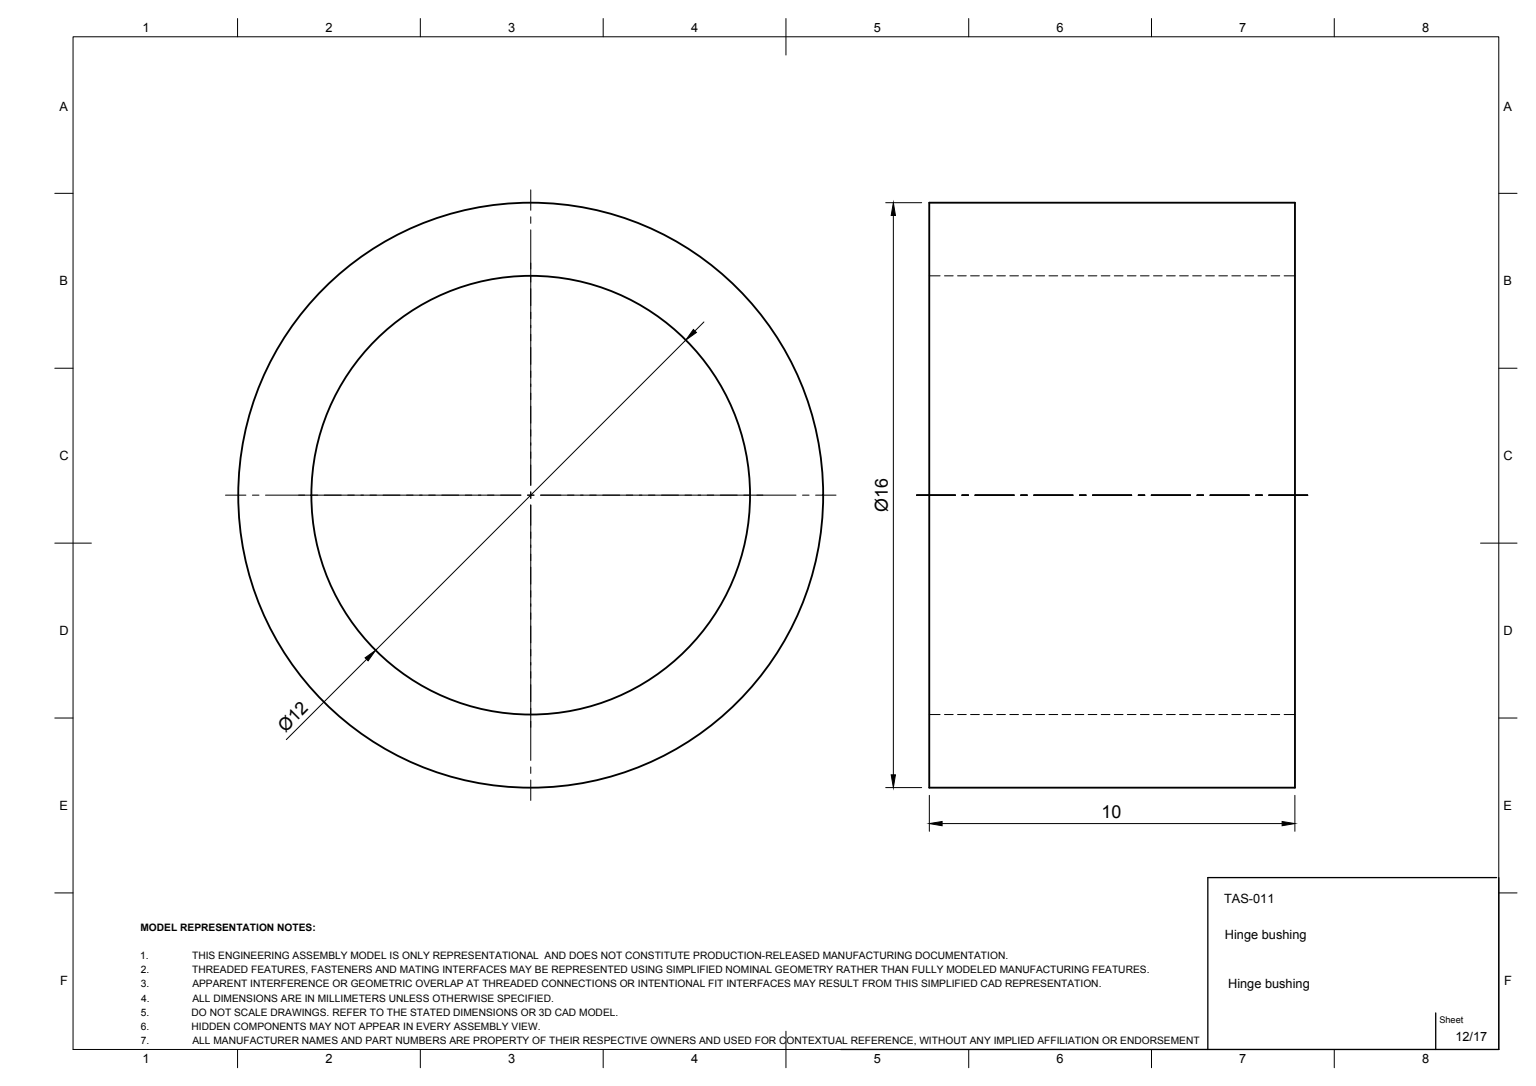
ISO-10303-21;
HEADER;
/* Generated by software containing ST-Developer
 * from STEP Tools, Inc. (www.steptools.com) 
 */

FILE_DESCRIPTION(
/* description */ (
'Independent manual bench leaf bending machine,200mm work width. Fabri
cated welded frame and folding leaf, repeated bushed and fully retaine
d hinge hardware, two handles with bonded grips, beveled clamping beam
 and modeledM12 clamp screws.2mm omitted-workpiece assembly reference 
gap, not a capacity claim. Native135deg hinge travel. Weld sizing, pro
duction fits, material condition, bending capacity, strength and life 
unassigned.'),
/* implementation_level */ '2;1');

FILE_NAME(
/* name */ 'Hinge bushing.step',
/* time_stamp */ '2026-11-14T09:11:34-08:00',
/* author */ (''),
/* organization */ (''),
/* preprocessor_version */ 'ST-DEVELOPER v20.2',
/* originating_system */ 'Autodesk Translation Framework v15.17.0.0',
/* authorisation */ '');

FILE_SCHEMA (('AUTOMOTIVE_DESIGN { 1 0 10303 214 3 1 1 }'));
ENDSEC;

DATA;
#10=MECHANICAL_DESIGN_GEOMETRIC_PRESENTATION_REPRESENTATION('',(#457),#37701);
#421=SHAPE_REPRESENTATION_RELATIONSHIP('SRR','None',#37790,#439);
#439=ADVANCED_BREP_SHAPE_REPRESENTATION('',(#475),#37694);
#457=STYLED_ITEM('',(#37880),#475);
#475=MANIFOLD_SOLID_BREP('Body1',#4155);
#508=FACE_BOUND('',#1018,.T.);
#509=FACE_BOUND('',#1020,.T.);
#578=PLANE('',#4610);
#579=PLANE('',#4611);
#777=FACE_OUTER_BOUND('',#1015,.T.);
#778=FACE_OUTER_BOUND('',#1016,.T.);
#779=FACE_OUTER_BOUND('',#1017,.T.);
#780=FACE_OUTER_BOUND('',#1019,.T.);
#1015=EDGE_LOOP('',(#3697,#3698,#3699,#3700));
#1016=EDGE_LOOP('',(#3701,#3702,#3703,#3704));
#1017=EDGE_LOOP('',(#3705));
#1018=EDGE_LOOP('',(#3706));
#1019=EDGE_LOOP('',(#3707));
#1020=EDGE_LOOP('',(#3708));
#1278=LINE('',#37494,#1527);
#1279=LINE('',#37500,#1528);
#1527=VECTOR('',#5415,6.);
#1528=VECTOR('',#5422,8.);
#1611=CIRCLE('',#4605,6.);
#1612=CIRCLE('',#4606,6.);
#1613=CIRCLE('',#4608,8.);
#1614=CIRCLE('',#4609,8.);
#2015=VERTEX_POINT('',#37491);
#2016=VERTEX_POINT('',#37493);
#2017=VERTEX_POINT('',#37497);
#2018=VERTEX_POINT('',#37499);
#2582=EDGE_CURVE('',#2015,#2015,#1611,.T.);
#2583=EDGE_CURVE('',#2015,#2016,#1278,.T.);
#2584=EDGE_CURVE('',#2016,#2016,#1612,.T.);
#2585=EDGE_CURVE('',#2017,#2017,#1613,.T.);
#2586=EDGE_CURVE('',#2017,#2018,#1279,.T.);
#2587=EDGE_CURVE('',#2018,#2018,#1614,.T.);
#3697=ORIENTED_EDGE('',*,*,#2582,.T.);
#3698=ORIENTED_EDGE('',*,*,#2583,.T.);
#3699=ORIENTED_EDGE('',*,*,#2584,.F.);
#3700=ORIENTED_EDGE('',*,*,#2583,.F.);
#3701=ORIENTED_EDGE('',*,*,#2585,.F.);
#3702=ORIENTED_EDGE('',*,*,#2586,.T.);
#3703=ORIENTED_EDGE('',*,*,#2587,.T.);
#3704=ORIENTED_EDGE('',*,*,#2586,.F.);
#3705=ORIENTED_EDGE('',*,*,#2585,.T.);
#3706=ORIENTED_EDGE('',*,*,#2584,.T.);
#3707=ORIENTED_EDGE('',*,*,#2587,.F.);
#3708=ORIENTED_EDGE('',*,*,#2582,.F.);
#3919=CYLINDRICAL_SURFACE('',#4604,6.);
#3920=CYLINDRICAL_SURFACE('',#4607,8.);
#4107=ADVANCED_FACE('',(#777),#3919,.F.);
#4108=ADVANCED_FACE('',(#778),#3920,.T.);
#4109=ADVANCED_FACE('',(#779,#508),#578,.T.);
#4110=ADVANCED_FACE('',(#780,#509),#579,.F.);
#4155=CLOSED_SHELL('',(#4107,#4108,#4109,#4110));
#4603=AXIS2_PLACEMENT_3D('',#37489,#5409,#5410);
#4604=AXIS2_PLACEMENT_3D('',#37490,#5411,#5412);
#4605=AXIS2_PLACEMENT_3D('',#37492,#5413,#5414);
#4606=AXIS2_PLACEMENT_3D('',#37495,#5416,#5417);
#4607=AXIS2_PLACEMENT_3D('',#37496,#5418,#5419);
#4608=AXIS2_PLACEMENT_3D('',#37498,#5420,#5421);
#4609=AXIS2_PLACEMENT_3D('',#37501,#5423,#5424);
#4610=AXIS2_PLACEMENT_3D('',#37502,#5425,#5426);
#4611=AXIS2_PLACEMENT_3D('',#37503,#5427,#5428);
#5409=DIRECTION('axis',(0.,0.,1.));
#5410=DIRECTION('refdir',(1.,0.,0.));
#5411=DIRECTION('center_axis',(0.,0.,1.));
#5412=DIRECTION('ref_axis',(1.,0.,0.));
#5413=DIRECTION('center_axis',(0.,0.,-1.));
#5414=DIRECTION('ref_axis',(1.,0.,0.));
#5415=DIRECTION('',(0.,0.,1.));
#5416=DIRECTION('center_axis',(0.,0.,-1.));
#5417=DIRECTION('ref_axis',(1.,0.,0.));
#5418=DIRECTION('center_axis',(0.,0.,1.));
#5419=DIRECTION('ref_axis',(1.,0.,0.));
#5420=DIRECTION('center_axis',(0.,0.,1.));
#5421=DIRECTION('ref_axis',(1.,0.,0.));
#5422=DIRECTION('',(0.,0.,-1.));
#5423=DIRECTION('center_axis',(0.,0.,1.));
#5424=DIRECTION('ref_axis',(1.,0.,0.));
#5425=DIRECTION('center_axis',(0.,0.,1.));
#5426=DIRECTION('ref_axis',(1.,0.,0.));
#5427=DIRECTION('center_axis',(0.,0.,1.));
#5428=DIRECTION('ref_axis',(1.,0.,0.));
#37489=CARTESIAN_POINT('',(0.,0.,0.));
#37490=CARTESIAN_POINT('Origin',(0.,0.,0.));
#37491=CARTESIAN_POINT('',(-6.,-7.34788079488412E-16,0.));
#37492=CARTESIAN_POINT('Origin',(0.,0.,0.));
#37493=CARTESIAN_POINT('',(-6.,-7.34788079488412E-16,10.));
#37494=CARTESIAN_POINT('',(-6.,-7.34788079488412E-16,0.));
#37495=CARTESIAN_POINT('Origin',(0.,0.,10.));
#37496=CARTESIAN_POINT('Origin',(0.,0.,0.));
#37497=CARTESIAN_POINT('',(-8.,-9.79717439317883E-16,10.));
#37498=CARTESIAN_POINT('Origin',(0.,0.,10.));
#37499=CARTESIAN_POINT('',(-8.,-9.79717439317883E-16,0.));
#37500=CARTESIAN_POINT('',(-8.,-9.79717439317883E-16,0.));
#37501=CARTESIAN_POINT('Origin',(0.,0.,0.));
#37502=CARTESIAN_POINT('Origin',(0.,0.,10.));
#37503=CARTESIAN_POINT('Origin',(0.,0.,0.));
#37674=UNCERTAINTY_MEASURE_WITH_UNIT(LENGTH_MEASURE(0.01),#37702,
'DISTANCE_ACCURACY_VALUE',
'Maximum model space distance between geometric entities at asserted c
onnectivities');
#37681=UNCERTAINTY_MEASURE_WITH_UNIT(LENGTH_MEASURE(0.01),#37702,
'DISTANCE_ACCURACY_VALUE',
'Maximum model space distance between geometric entities at asserted c
onnectivities');
#37694=(
GEOMETRIC_REPRESENTATION_CONTEXT(3)
GLOBAL_UNCERTAINTY_ASSIGNED_CONTEXT((#37674))
GLOBAL_UNIT_ASSIGNED_CONTEXT((#37702,#37704,#37705))
REPRESENTATION_CONTEXT('','3D')
);
#37701=(
GEOMETRIC_REPRESENTATION_CONTEXT(3)
GLOBAL_UNCERTAINTY_ASSIGNED_CONTEXT((#37681))
GLOBAL_UNIT_ASSIGNED_CONTEXT((#37702,#37704,#37705))
REPRESENTATION_CONTEXT('','3D')
);
#37702=(
LENGTH_UNIT()
NAMED_UNIT(*)
SI_UNIT(.MILLI.,.METRE.)
);
#37704=(
NAMED_UNIT(*)
PLANE_ANGLE_UNIT()
SI_UNIT($,.RADIAN.)
);
#37705=(
NAMED_UNIT(*)
SI_UNIT($,.STERADIAN.)
SOLID_ANGLE_UNIT()
);
#37718=SHAPE_DEFINITION_REPRESENTATION(#37737,#37790);
#37737=PRODUCT_DEFINITION_SHAPE('',$,#37810);
#37790=SHAPE_REPRESENTATION('',(#4603),#37694);
#37797=PRODUCT_DEFINITION_CONTEXT('part definition',#37856,'design');
#37810=PRODUCT_DEFINITION('Hinge bushing','Hinge bushing',#37829,#37797);
#37829=PRODUCT_DEFINITION_FORMATION('',$,#37870);
#37856=APPLICATION_CONTEXT(
'Core Data for Automotive Mechanical Design Process');
#37857=PRODUCT_CONTEXT('part definition',#37856,'mechanical');
#37870=PRODUCT('Hinge bushing','Hinge bushing',$,(#37857));
#37880=PRESENTATION_STYLE_ASSIGNMENT((#37888));
#37888=SURFACE_STYLE_USAGE(.BOTH.,#37896);
#37896=SURFACE_SIDE_STYLE('',(#37904));
#37904=SURFACE_STYLE_FILL_AREA(#37912);
#37912=FILL_AREA_STYLE('Opaque(185,192,202)',(#37920));
#37920=FILL_AREA_STYLE_COLOUR('Opaque(185,192,202)',#37928);
#37928=COLOUR_RGB('Opaque(185,192,202)',0.725490196078431,0.752941176470588,
0.792156862745098);
ENDSEC;
END-ISO-10303-21;
